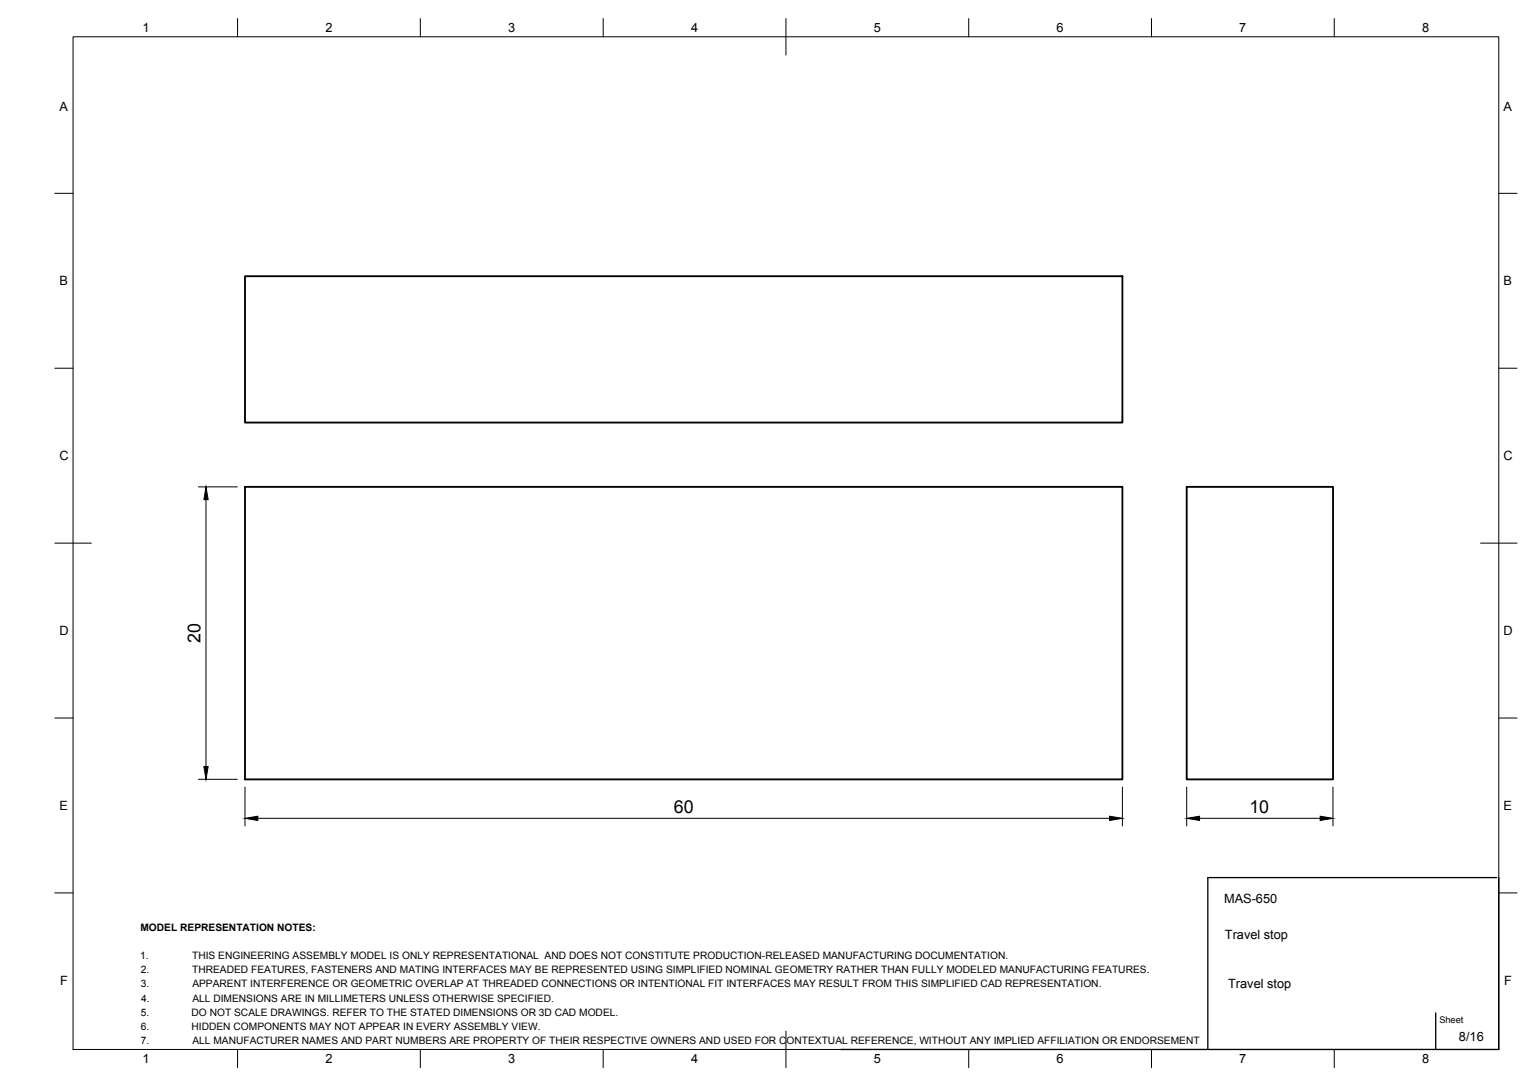
ISO-10303-21;
HEADER;
/* Generated by software containing ST-Developer
 * from STEP Tools, Inc. (www.steptools.com) 
 */

FILE_DESCRIPTION(
/* description */ ('Independent manual traversing gantry with native reusable aluminum pr
ofiles,180mm captured carriage travel, four bronze-bushed rollers, lin
ked ideal rolling motion, bonded acetal lateral guides, positive welde
d end stops and fully retained axle stacks. Editable native profile cu
t lengths220/400mm. Tool attachments viaM6 bridge-plate taps; mounted 
tool outside assembly. Welds, anchors, adhesives, fits, traction, load
/speed/structural/life ratings unassigned.'),
/* implementation_level */ '2;1');

FILE_NAME(
/* name */ 'Travel stop.step',
/* time_stamp */ '2026-11-09T20:04:38-08:00',
/* author */ (''),
/* organization */ (''),
/* preprocessor_version */ 'ST-DEVELOPER v20.2',
/* originating_system */ 'Autodesk Translation Framework v15.17.0.0',
/* authorisation */ '');

FILE_SCHEMA (('AUTOMOTIVE_DESIGN { 1 0 10303 214 3 1 1 }'));
ENDSEC;

DATA;
#10=MECHANICAL_DESIGN_GEOMETRIC_PRESENTATION_REPRESENTATION('',(#476),#13231);
#444=SHAPE_REPRESENTATION_RELATIONSHIP('SRR','None',#13333,#460);
#460=ADVANCED_BREP_SHAPE_REPRESENTATION('',(#492),#13220);
#476=STYLED_ITEM('',(#13422),#492);
#492=MANIFOLD_SOLID_BREP('Body1',#4156);
#590=PLANE('',#4461);
#591=PLANE('',#4462);
#592=PLANE('',#4463);
#593=PLANE('',#4464);
#594=PLANE('',#4465);
#595=PLANE('',#4466);
#695=FACE_OUTER_BOUND('',#936,.T.);
#696=FACE_OUTER_BOUND('',#937,.T.);
#697=FACE_OUTER_BOUND('',#938,.T.);
#698=FACE_OUTER_BOUND('',#939,.T.);
#699=FACE_OUTER_BOUND('',#940,.T.);
#700=FACE_OUTER_BOUND('',#941,.T.);
#936=EDGE_LOOP('',(#2994,#2995,#2996,#2997));
#937=EDGE_LOOP('',(#2998,#2999,#3000,#3001));
#938=EDGE_LOOP('',(#3002,#3003,#3004,#3005));
#939=EDGE_LOOP('',(#3006,#3007,#3008,#3009));
#940=EDGE_LOOP('',(#3010,#3011,#3012,#3013));
#941=EDGE_LOOP('',(#3014,#3015,#3016,#3017));
#1232=LINE('',#6111,#1494);
#1233=LINE('',#6113,#1495);
#1234=LINE('',#6115,#1496);
#1235=LINE('',#6116,#1497);
#1236=LINE('',#6119,#1498);
#1237=LINE('',#6121,#1499);
#1238=LINE('',#6122,#1500);
#1239=LINE('',#6125,#1501);
#1240=LINE('',#6127,#1502);
#1241=LINE('',#6128,#1503);
#1242=LINE('',#6130,#1504);
#1243=LINE('',#6131,#1505);
#1494=VECTOR('',#5079,10.);
#1495=VECTOR('',#5080,10.);
#1496=VECTOR('',#5081,10.);
#1497=VECTOR('',#5082,10.);
#1498=VECTOR('',#5085,10.);
#1499=VECTOR('',#5086,10.);
#1500=VECTOR('',#5087,10.);
#1501=VECTOR('',#5090,10.);
#1502=VECTOR('',#5091,10.);
#1503=VECTOR('',#5092,10.);
#1504=VECTOR('',#5095,10.);
#1505=VECTOR('',#5096,10.);
#1856=VERTEX_POINT('',#6109);
#1857=VERTEX_POINT('',#6110);
#1858=VERTEX_POINT('',#6112);
#1859=VERTEX_POINT('',#6114);
#1860=VERTEX_POINT('',#6118);
#1861=VERTEX_POINT('',#6120);
#1862=VERTEX_POINT('',#6124);
#1863=VERTEX_POINT('',#6126);
#2280=EDGE_CURVE('',#1856,#1857,#1232,.T.);
#2281=EDGE_CURVE('',#1857,#1858,#1233,.T.);
#2282=EDGE_CURVE('',#1859,#1858,#1234,.T.);
#2283=EDGE_CURVE('',#1856,#1859,#1235,.T.);
#2284=EDGE_CURVE('',#1860,#1856,#1236,.T.);
#2285=EDGE_CURVE('',#1861,#1859,#1237,.T.);
#2286=EDGE_CURVE('',#1860,#1861,#1238,.T.);
#2287=EDGE_CURVE('',#1862,#1860,#1239,.T.);
#2288=EDGE_CURVE('',#1863,#1861,#1240,.T.);
#2289=EDGE_CURVE('',#1862,#1863,#1241,.T.);
#2290=EDGE_CURVE('',#1857,#1862,#1242,.T.);
#2291=EDGE_CURVE('',#1858,#1863,#1243,.T.);
#2994=ORIENTED_EDGE('',*,*,#2280,.T.);
#2995=ORIENTED_EDGE('',*,*,#2281,.T.);
#2996=ORIENTED_EDGE('',*,*,#2282,.F.);
#2997=ORIENTED_EDGE('',*,*,#2283,.F.);
#2998=ORIENTED_EDGE('',*,*,#2284,.T.);
#2999=ORIENTED_EDGE('',*,*,#2283,.T.);
#3000=ORIENTED_EDGE('',*,*,#2285,.F.);
#3001=ORIENTED_EDGE('',*,*,#2286,.F.);
#3002=ORIENTED_EDGE('',*,*,#2287,.T.);
#3003=ORIENTED_EDGE('',*,*,#2286,.T.);
#3004=ORIENTED_EDGE('',*,*,#2288,.F.);
#3005=ORIENTED_EDGE('',*,*,#2289,.F.);
#3006=ORIENTED_EDGE('',*,*,#2290,.T.);
#3007=ORIENTED_EDGE('',*,*,#2289,.T.);
#3008=ORIENTED_EDGE('',*,*,#2291,.F.);
#3009=ORIENTED_EDGE('',*,*,#2281,.F.);
#3010=ORIENTED_EDGE('',*,*,#2291,.T.);
#3011=ORIENTED_EDGE('',*,*,#2288,.T.);
#3012=ORIENTED_EDGE('',*,*,#2285,.T.);
#3013=ORIENTED_EDGE('',*,*,#2282,.T.);
#3014=ORIENTED_EDGE('',*,*,#2290,.F.);
#3015=ORIENTED_EDGE('',*,*,#2280,.F.);
#3016=ORIENTED_EDGE('',*,*,#2284,.F.);
#3017=ORIENTED_EDGE('',*,*,#2287,.F.);
#3992=ADVANCED_FACE('',(#695),#590,.T.);
#3993=ADVANCED_FACE('',(#696),#591,.T.);
#3994=ADVANCED_FACE('',(#697),#592,.T.);
#3995=ADVANCED_FACE('',(#698),#593,.T.);
#3996=ADVANCED_FACE('',(#699),#594,.T.);
#3997=ADVANCED_FACE('',(#700),#595,.F.);
#4156=CLOSED_SHELL('',(#3992,#3993,#3994,#3995,#3996,#3997));
#4460=AXIS2_PLACEMENT_3D('',#6107,#5075,#5076);
#4461=AXIS2_PLACEMENT_3D('',#6108,#5077,#5078);
#4462=AXIS2_PLACEMENT_3D('',#6117,#5083,#5084);
#4463=AXIS2_PLACEMENT_3D('',#6123,#5088,#5089);
#4464=AXIS2_PLACEMENT_3D('',#6129,#5093,#5094);
#4465=AXIS2_PLACEMENT_3D('',#6132,#5097,#5098);
#4466=AXIS2_PLACEMENT_3D('',#6133,#5099,#5100);
#5075=DIRECTION('axis',(0.,0.,1.));
#5076=DIRECTION('refdir',(1.,0.,0.));
#5077=DIRECTION('center_axis',(0.,1.,0.));
#5078=DIRECTION('ref_axis',(-1.,0.,0.));
#5079=DIRECTION('',(-1.,0.,0.));
#5080=DIRECTION('',(0.,0.,1.));
#5081=DIRECTION('',(-1.,0.,0.));
#5082=DIRECTION('',(0.,0.,1.));
#5083=DIRECTION('center_axis',(1.,0.,0.));
#5084=DIRECTION('ref_axis',(0.,1.,0.));
#5085=DIRECTION('',(0.,1.,0.));
#5086=DIRECTION('',(0.,1.,0.));
#5087=DIRECTION('',(0.,0.,1.));
#5088=DIRECTION('center_axis',(0.,-1.,0.));
#5089=DIRECTION('ref_axis',(1.,0.,0.));
#5090=DIRECTION('',(1.,0.,0.));
#5091=DIRECTION('',(1.,0.,0.));
#5092=DIRECTION('',(0.,0.,1.));
#5093=DIRECTION('center_axis',(-1.,0.,0.));
#5094=DIRECTION('ref_axis',(0.,-1.,0.));
#5095=DIRECTION('',(0.,-1.,0.));
#5096=DIRECTION('',(0.,-1.,0.));
#5097=DIRECTION('center_axis',(0.,0.,1.));
#5098=DIRECTION('ref_axis',(1.,0.,0.));
#5099=DIRECTION('center_axis',(0.,0.,1.));
#5100=DIRECTION('ref_axis',(1.,0.,0.));
#6107=CARTESIAN_POINT('',(0.,0.,0.));
#6108=CARTESIAN_POINT('Origin',(5.,30.,0.));
#6109=CARTESIAN_POINT('',(5.,30.,0.));
#6110=CARTESIAN_POINT('',(-5.,30.,0.));
#6111=CARTESIAN_POINT('',(5.,30.,0.));
#6112=CARTESIAN_POINT('',(-5.,30.,20.));
#6113=CARTESIAN_POINT('',(-5.,30.,0.));
#6114=CARTESIAN_POINT('',(5.,30.,20.));
#6115=CARTESIAN_POINT('',(5.,30.,20.));
#6116=CARTESIAN_POINT('',(5.,30.,0.));
#6117=CARTESIAN_POINT('Origin',(5.,-30.,0.));
#6118=CARTESIAN_POINT('',(5.,-30.,0.));
#6119=CARTESIAN_POINT('',(5.,-30.,0.));
#6120=CARTESIAN_POINT('',(5.,-30.,20.));
#6121=CARTESIAN_POINT('',(5.,-30.,20.));
#6122=CARTESIAN_POINT('',(5.,-30.,0.));
#6123=CARTESIAN_POINT('Origin',(-5.,-30.,0.));
#6124=CARTESIAN_POINT('',(-5.,-30.,0.));
#6125=CARTESIAN_POINT('',(-5.,-30.,0.));
#6126=CARTESIAN_POINT('',(-5.,-30.,20.));
#6127=CARTESIAN_POINT('',(-5.,-30.,20.));
#6128=CARTESIAN_POINT('',(-5.,-30.,0.));
#6129=CARTESIAN_POINT('Origin',(-5.,30.,0.));
#6130=CARTESIAN_POINT('',(-5.,30.,0.));
#6131=CARTESIAN_POINT('',(-5.,30.,20.));
#6132=CARTESIAN_POINT('Origin',(0.,0.,20.));
#6133=CARTESIAN_POINT('Origin',(0.,0.,0.));
#13202=UNCERTAINTY_MEASURE_WITH_UNIT(LENGTH_MEASURE(0.01),#13232,
'DISTANCE_ACCURACY_VALUE',
'Maximum model space distance between geometric entities at asserted c
onnectivities');
#13213=UNCERTAINTY_MEASURE_WITH_UNIT(LENGTH_MEASURE(0.01),#13232,
'DISTANCE_ACCURACY_VALUE',
'Maximum model space distance between geometric entities at asserted c
onnectivities');
#13220=(
GEOMETRIC_REPRESENTATION_CONTEXT(3)
GLOBAL_UNCERTAINTY_ASSIGNED_CONTEXT((#13202))
GLOBAL_UNIT_ASSIGNED_CONTEXT((#13232,#13234,#13235))
REPRESENTATION_CONTEXT('','3D')
);
#13231=(
GEOMETRIC_REPRESENTATION_CONTEXT(3)
GLOBAL_UNCERTAINTY_ASSIGNED_CONTEXT((#13213))
GLOBAL_UNIT_ASSIGNED_CONTEXT((#13232,#13234,#13235))
REPRESENTATION_CONTEXT('','3D')
);
#13232=(
LENGTH_UNIT()
NAMED_UNIT(*)
SI_UNIT(.MILLI.,.METRE.)
);
#13234=(
NAMED_UNIT(*)
PLANE_ANGLE_UNIT()
SI_UNIT($,.RADIAN.)
);
#13235=(
NAMED_UNIT(*)
SI_UNIT($,.STERADIAN.)
SOLID_ANGLE_UNIT()
);
#13242=SHAPE_DEFINITION_REPRESENTATION(#13259,#13333);
#13259=PRODUCT_DEFINITION_SHAPE('',$,#13351);
#13333=SHAPE_REPRESENTATION('',(#4460),#13220);
#13344=PRODUCT_DEFINITION_CONTEXT('part definition',#13397,'design');
#13351=PRODUCT_DEFINITION('Travel stop','Travel stop',#13368,#13344);
#13368=PRODUCT_DEFINITION_FORMATION('',$,#13405);
#13397=APPLICATION_CONTEXT(
'Core Data for Automotive Mechanical Design Process');
#13398=PRODUCT_CONTEXT('part definition',#13397,'mechanical');
#13405=PRODUCT('Travel stop','Travel stop','Travel stop',(#13398));
#13422=PRESENTATION_STYLE_ASSIGNMENT((#13436));
#13436=SURFACE_STYLE_USAGE(.BOTH.,#13450);
#13450=SURFACE_SIDE_STYLE('',(#13464));
#13464=SURFACE_STYLE_FILL_AREA(#13478);
#13478=FILL_AREA_STYLE('Gray',(#13492));
#13492=FILL_AREA_STYLE_COLOUR('Gray',#13506);
#13506=COLOUR_RGB('Gray',0.407843137254902,0.447058823529412,0.498039215686275);
ENDSEC;
END-ISO-10303-21;
